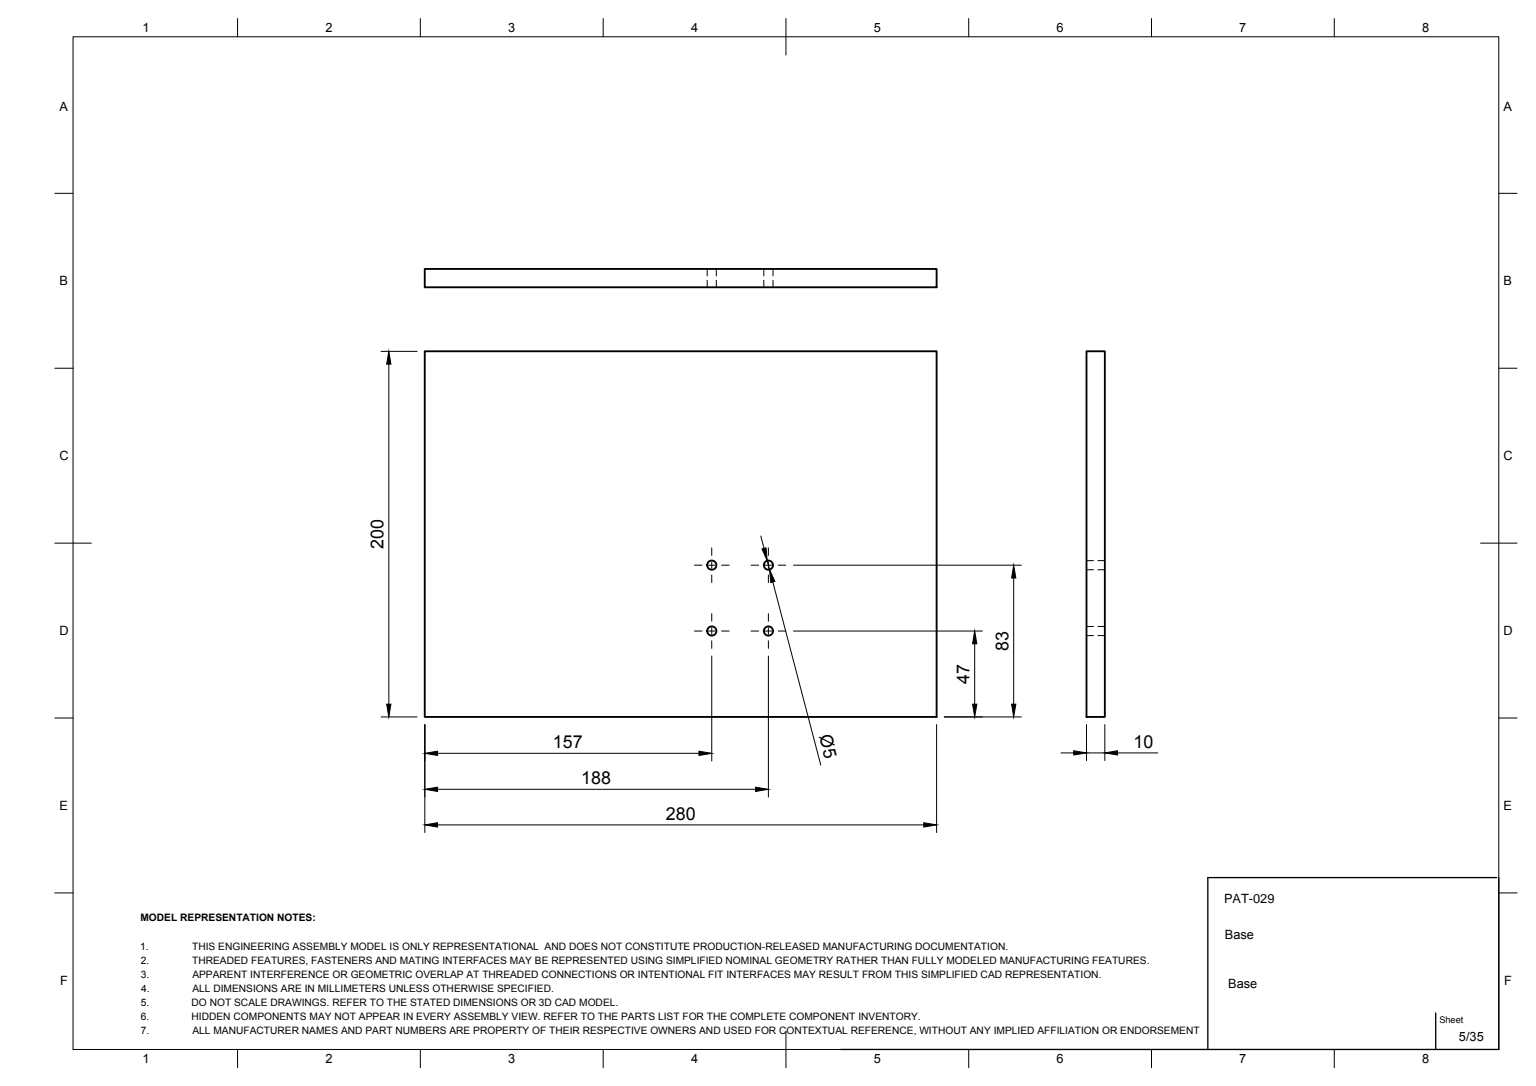
ISO-10303-21;
HEADER;
/* Generated by software containing ST-Developer
 * from STEP Tools, Inc. (www.steptools.com) 
 */

FILE_DESCRIPTION(
/* description */ ('Door-style hinge test fixture with detent'),
/* implementation_level */ '2;1');

FILE_NAME(
/* name */ 'Base.step',
/* time_stamp */ '2026-10-28T03:24:57-07:00',
/* author */ (''),
/* organization */ (''),
/* preprocessor_version */ 'ST-DEVELOPER v20.2',
/* originating_system */ 'Autodesk Translation Framework v15.17.0.0',
/* authorisation */ '');

FILE_SCHEMA (('AUTOMOTIVE_DESIGN { 1 0 10303 214 3 1 1 }'));
ENDSEC;

DATA;
#10=MECHANICAL_DESIGN_GEOMETRIC_PRESENTATION_REPRESENTATION('',(#322),#9813);
#260=SHAPE_REPRESENTATION_RELATIONSHIP('SRR','None',#9937,#291);
#291=ADVANCED_BREP_SHAPE_REPRESENTATION('',(#362),#9780);
#322=STYLED_ITEM('',(#10162),#362);
#362=MANIFOLD_SOLID_BREP('Body1',#4753);
#399=FACE_BOUND('',#957,.T.);
#400=FACE_BOUND('',#958,.T.);
#401=FACE_BOUND('',#959,.T.);
#402=FACE_BOUND('',#960,.T.);
#403=FACE_BOUND('',#962,.T.);
#404=FACE_BOUND('',#963,.T.);
#405=FACE_BOUND('',#964,.T.);
#406=FACE_BOUND('',#965,.T.);
#500=PLANE('',#5153);
#501=PLANE('',#5154);
#502=PLANE('',#5155);
#503=PLANE('',#5156);
#504=PLANE('',#5157);
#505=PLANE('',#5158);
#663=FACE_OUTER_BOUND('',#948,.T.);
#664=FACE_OUTER_BOUND('',#949,.T.);
#665=FACE_OUTER_BOUND('',#950,.T.);
#666=FACE_OUTER_BOUND('',#951,.T.);
#667=FACE_OUTER_BOUND('',#952,.T.);
#668=FACE_OUTER_BOUND('',#953,.T.);
#669=FACE_OUTER_BOUND('',#954,.T.);
#670=FACE_OUTER_BOUND('',#955,.T.);
#671=FACE_OUTER_BOUND('',#956,.T.);
#672=FACE_OUTER_BOUND('',#961,.T.);
#948=EDGE_LOOP('',(#3207,#3208,#3209,#3210));
#949=EDGE_LOOP('',(#3211,#3212,#3213,#3214));
#950=EDGE_LOOP('',(#3215,#3216,#3217,#3218));
#951=EDGE_LOOP('',(#3219,#3220,#3221,#3222));
#952=EDGE_LOOP('',(#3223,#3224,#3225,#3226));
#953=EDGE_LOOP('',(#3227,#3228,#3229,#3230));
#954=EDGE_LOOP('',(#3231,#3232,#3233,#3234));
#955=EDGE_LOOP('',(#3235,#3236,#3237,#3238));
#956=EDGE_LOOP('',(#3239,#3240,#3241,#3242));
#957=EDGE_LOOP('',(#3243));
#958=EDGE_LOOP('',(#3244));
#959=EDGE_LOOP('',(#3245));
#960=EDGE_LOOP('',(#3246));
#961=EDGE_LOOP('',(#3247,#3248,#3249,#3250));
#962=EDGE_LOOP('',(#3251));
#963=EDGE_LOOP('',(#3252));
#964=EDGE_LOOP('',(#3253));
#965=EDGE_LOOP('',(#3254));
#1334=LINE('',#7304,#1654);
#1335=LINE('',#7310,#1655);
#1336=LINE('',#7316,#1656);
#1337=LINE('',#7322,#1657);
#1338=LINE('',#7327,#1658);
#1339=LINE('',#7329,#1659);
#1340=LINE('',#7331,#1660);
#1341=LINE('',#7332,#1661);
#1342=LINE('',#7335,#1662);
#1343=LINE('',#7337,#1663);
#1344=LINE('',#7338,#1664);
#1345=LINE('',#7341,#1665);
#1346=LINE('',#7343,#1666);
#1347=LINE('',#7344,#1667);
#1348=LINE('',#7346,#1668);
#1349=LINE('',#7347,#1669);
#1654=VECTOR('',#5761,0.25);
#1655=VECTOR('',#5768,0.25);
#1656=VECTOR('',#5775,0.25);
#1657=VECTOR('',#5782,0.25);
#1658=VECTOR('',#5787,1.);
#1659=VECTOR('',#5788,1.);
#1660=VECTOR('',#5789,1.);
#1661=VECTOR('',#5790,1.);
#1662=VECTOR('',#5793,1.);
#1663=VECTOR('',#5794,1.);
#1664=VECTOR('',#5795,1.);
#1665=VECTOR('',#5798,1.);
#1666=VECTOR('',#5799,1.);
#1667=VECTOR('',#5800,1.);
#1668=VECTOR('',#5803,1.);
#1669=VECTOR('',#5804,1.);
#1974=CIRCLE('',#5142,0.25);
#1975=CIRCLE('',#5143,0.25);
#1976=CIRCLE('',#5145,0.25);
#1977=CIRCLE('',#5146,0.25);
#1978=CIRCLE('',#5148,0.25);
#1979=CIRCLE('',#5149,0.25);
#1980=CIRCLE('',#5151,0.25);
#1981=CIRCLE('',#5152,0.25);
#2221=VERTEX_POINT('',#7301);
#2222=VERTEX_POINT('',#7303);
#2223=VERTEX_POINT('',#7307);
#2224=VERTEX_POINT('',#7309);
#2225=VERTEX_POINT('',#7313);
#2226=VERTEX_POINT('',#7315);
#2227=VERTEX_POINT('',#7319);
#2228=VERTEX_POINT('',#7321);
#2229=VERTEX_POINT('',#7325);
#2230=VERTEX_POINT('',#7326);
#2231=VERTEX_POINT('',#7328);
#2232=VERTEX_POINT('',#7330);
#2233=VERTEX_POINT('',#7334);
#2234=VERTEX_POINT('',#7336);
#2235=VERTEX_POINT('',#7340);
#2236=VERTEX_POINT('',#7342);
#2620=EDGE_CURVE('',#2221,#2221,#1974,.T.);
#2621=EDGE_CURVE('',#2221,#2222,#1334,.T.);
#2622=EDGE_CURVE('',#2222,#2222,#1975,.T.);
#2623=EDGE_CURVE('',#2223,#2223,#1976,.T.);
#2624=EDGE_CURVE('',#2223,#2224,#1335,.T.);
#2625=EDGE_CURVE('',#2224,#2224,#1977,.T.);
#2626=EDGE_CURVE('',#2225,#2225,#1978,.T.);
#2627=EDGE_CURVE('',#2225,#2226,#1336,.T.);
#2628=EDGE_CURVE('',#2226,#2226,#1979,.T.);
#2629=EDGE_CURVE('',#2227,#2227,#1980,.T.);
#2630=EDGE_CURVE('',#2227,#2228,#1337,.T.);
#2631=EDGE_CURVE('',#2228,#2228,#1981,.T.);
#2632=EDGE_CURVE('',#2229,#2230,#1338,.T.);
#2633=EDGE_CURVE('',#2230,#2231,#1339,.T.);
#2634=EDGE_CURVE('',#2232,#2231,#1340,.T.);
#2635=EDGE_CURVE('',#2229,#2232,#1341,.T.);
#2636=EDGE_CURVE('',#2233,#2229,#1342,.T.);
#2637=EDGE_CURVE('',#2234,#2232,#1343,.T.);
#2638=EDGE_CURVE('',#2233,#2234,#1344,.T.);
#2639=EDGE_CURVE('',#2235,#2233,#1345,.T.);
#2640=EDGE_CURVE('',#2236,#2234,#1346,.T.);
#2641=EDGE_CURVE('',#2235,#2236,#1347,.T.);
#2642=EDGE_CURVE('',#2230,#2235,#1348,.T.);
#2643=EDGE_CURVE('',#2231,#2236,#1349,.T.);
#3207=ORIENTED_EDGE('',*,*,#2620,.F.);
#3208=ORIENTED_EDGE('',*,*,#2621,.T.);
#3209=ORIENTED_EDGE('',*,*,#2622,.F.);
#3210=ORIENTED_EDGE('',*,*,#2621,.F.);
#3211=ORIENTED_EDGE('',*,*,#2623,.F.);
#3212=ORIENTED_EDGE('',*,*,#2624,.T.);
#3213=ORIENTED_EDGE('',*,*,#2625,.F.);
#3214=ORIENTED_EDGE('',*,*,#2624,.F.);
#3215=ORIENTED_EDGE('',*,*,#2626,.F.);
#3216=ORIENTED_EDGE('',*,*,#2627,.T.);
#3217=ORIENTED_EDGE('',*,*,#2628,.F.);
#3218=ORIENTED_EDGE('',*,*,#2627,.F.);
#3219=ORIENTED_EDGE('',*,*,#2629,.F.);
#3220=ORIENTED_EDGE('',*,*,#2630,.T.);
#3221=ORIENTED_EDGE('',*,*,#2631,.F.);
#3222=ORIENTED_EDGE('',*,*,#2630,.F.);
#3223=ORIENTED_EDGE('',*,*,#2632,.T.);
#3224=ORIENTED_EDGE('',*,*,#2633,.T.);
#3225=ORIENTED_EDGE('',*,*,#2634,.F.);
#3226=ORIENTED_EDGE('',*,*,#2635,.F.);
#3227=ORIENTED_EDGE('',*,*,#2636,.T.);
#3228=ORIENTED_EDGE('',*,*,#2635,.T.);
#3229=ORIENTED_EDGE('',*,*,#2637,.F.);
#3230=ORIENTED_EDGE('',*,*,#2638,.F.);
#3231=ORIENTED_EDGE('',*,*,#2639,.T.);
#3232=ORIENTED_EDGE('',*,*,#2638,.T.);
#3233=ORIENTED_EDGE('',*,*,#2640,.F.);
#3234=ORIENTED_EDGE('',*,*,#2641,.F.);
#3235=ORIENTED_EDGE('',*,*,#2642,.T.);
#3236=ORIENTED_EDGE('',*,*,#2641,.T.);
#3237=ORIENTED_EDGE('',*,*,#2643,.F.);
#3238=ORIENTED_EDGE('',*,*,#2633,.F.);
#3239=ORIENTED_EDGE('',*,*,#2643,.T.);
#3240=ORIENTED_EDGE('',*,*,#2640,.T.);
#3241=ORIENTED_EDGE('',*,*,#2637,.T.);
#3242=ORIENTED_EDGE('',*,*,#2634,.T.);
#3243=ORIENTED_EDGE('',*,*,#2622,.T.);
#3244=ORIENTED_EDGE('',*,*,#2625,.T.);
#3245=ORIENTED_EDGE('',*,*,#2628,.T.);
#3246=ORIENTED_EDGE('',*,*,#2631,.T.);
#3247=ORIENTED_EDGE('',*,*,#2642,.F.);
#3248=ORIENTED_EDGE('',*,*,#2632,.F.);
#3249=ORIENTED_EDGE('',*,*,#2636,.F.);
#3250=ORIENTED_EDGE('',*,*,#2639,.F.);
#3251=ORIENTED_EDGE('',*,*,#2620,.T.);
#3252=ORIENTED_EDGE('',*,*,#2623,.T.);
#3253=ORIENTED_EDGE('',*,*,#2626,.T.);
#3254=ORIENTED_EDGE('',*,*,#2629,.T.);
#4381=CYLINDRICAL_SURFACE('',#5141,0.25);
#4382=CYLINDRICAL_SURFACE('',#5144,0.25);
#4383=CYLINDRICAL_SURFACE('',#5147,0.25);
#4384=CYLINDRICAL_SURFACE('',#5150,0.25);
#4468=ADVANCED_FACE('',(#663),#4381,.F.);
#4469=ADVANCED_FACE('',(#664),#4382,.F.);
#4470=ADVANCED_FACE('',(#665),#4383,.F.);
#4471=ADVANCED_FACE('',(#666),#4384,.F.);
#4472=ADVANCED_FACE('',(#667),#500,.T.);
#4473=ADVANCED_FACE('',(#668),#501,.T.);
#4474=ADVANCED_FACE('',(#669),#502,.T.);
#4475=ADVANCED_FACE('',(#670),#503,.T.);
#4476=ADVANCED_FACE('',(#671,#399,#400,#401,#402),#504,.T.);
#4477=ADVANCED_FACE('',(#672,#403,#404,#405,#406),#505,.F.);
#4753=CLOSED_SHELL('',(#4468,#4469,#4470,#4471,#4472,#4473,#4474,#4475,
#4476,#4477));
#5140=AXIS2_PLACEMENT_3D('',#7299,#5755,#5756);
#5141=AXIS2_PLACEMENT_3D('',#7300,#5757,#5758);
#5142=AXIS2_PLACEMENT_3D('',#7302,#5759,#5760);
#5143=AXIS2_PLACEMENT_3D('',#7305,#5762,#5763);
#5144=AXIS2_PLACEMENT_3D('',#7306,#5764,#5765);
#5145=AXIS2_PLACEMENT_3D('',#7308,#5766,#5767);
#5146=AXIS2_PLACEMENT_3D('',#7311,#5769,#5770);
#5147=AXIS2_PLACEMENT_3D('',#7312,#5771,#5772);
#5148=AXIS2_PLACEMENT_3D('',#7314,#5773,#5774);
#5149=AXIS2_PLACEMENT_3D('',#7317,#5776,#5777);
#5150=AXIS2_PLACEMENT_3D('',#7318,#5778,#5779);
#5151=AXIS2_PLACEMENT_3D('',#7320,#5780,#5781);
#5152=AXIS2_PLACEMENT_3D('',#7323,#5783,#5784);
#5153=AXIS2_PLACEMENT_3D('',#7324,#5785,#5786);
#5154=AXIS2_PLACEMENT_3D('',#7333,#5791,#5792);
#5155=AXIS2_PLACEMENT_3D('',#7339,#5796,#5797);
#5156=AXIS2_PLACEMENT_3D('',#7345,#5801,#5802);
#5157=AXIS2_PLACEMENT_3D('',#7348,#5805,#5806);
#5158=AXIS2_PLACEMENT_3D('',#7349,#5807,#5808);
#5755=DIRECTION('axis',(0.,0.,1.));
#5756=DIRECTION('refdir',(1.,0.,0.));
#5757=DIRECTION('center_axis',(0.,0.,1.));
#5758=DIRECTION('ref_axis',(1.,0.,0.));
#5759=DIRECTION('center_axis',(0.,0.,1.));
#5760=DIRECTION('ref_axis',(1.,0.,0.));
#5761=DIRECTION('',(0.,0.,1.));
#5762=DIRECTION('center_axis',(0.,0.,-1.));
#5763=DIRECTION('ref_axis',(1.,0.,0.));
#5764=DIRECTION('center_axis',(0.,0.,1.));
#5765=DIRECTION('ref_axis',(1.,0.,0.));
#5766=DIRECTION('center_axis',(0.,0.,1.));
#5767=DIRECTION('ref_axis',(1.,0.,0.));
#5768=DIRECTION('',(0.,0.,1.));
#5769=DIRECTION('center_axis',(0.,0.,-1.));
#5770=DIRECTION('ref_axis',(1.,0.,0.));
#5771=DIRECTION('center_axis',(0.,0.,1.));
#5772=DIRECTION('ref_axis',(1.,0.,0.));
#5773=DIRECTION('center_axis',(0.,0.,1.));
#5774=DIRECTION('ref_axis',(1.,0.,0.));
#5775=DIRECTION('',(0.,0.,1.));
#5776=DIRECTION('center_axis',(0.,0.,-1.));
#5777=DIRECTION('ref_axis',(1.,0.,0.));
#5778=DIRECTION('center_axis',(0.,0.,1.));
#5779=DIRECTION('ref_axis',(1.,0.,0.));
#5780=DIRECTION('center_axis',(0.,0.,1.));
#5781=DIRECTION('ref_axis',(1.,0.,0.));
#5782=DIRECTION('',(0.,0.,1.));
#5783=DIRECTION('center_axis',(0.,0.,-1.));
#5784=DIRECTION('ref_axis',(1.,0.,0.));
#5785=DIRECTION('center_axis',(0.,1.,0.));
#5786=DIRECTION('ref_axis',(-1.,0.,0.));
#5787=DIRECTION('',(-1.,0.,0.));
#5788=DIRECTION('',(0.,0.,1.));
#5789=DIRECTION('',(-1.,0.,0.));
#5790=DIRECTION('',(0.,0.,1.));
#5791=DIRECTION('center_axis',(1.,0.,0.));
#5792=DIRECTION('ref_axis',(0.,1.,0.));
#5793=DIRECTION('',(0.,1.,0.));
#5794=DIRECTION('',(0.,1.,0.));
#5795=DIRECTION('',(0.,0.,1.));
#5796=DIRECTION('center_axis',(0.,-1.,0.));
#5797=DIRECTION('ref_axis',(1.,0.,0.));
#5798=DIRECTION('',(1.,0.,0.));
#5799=DIRECTION('',(1.,0.,0.));
#5800=DIRECTION('',(0.,0.,1.));
#5801=DIRECTION('center_axis',(-1.,0.,0.));
#5802=DIRECTION('ref_axis',(0.,-1.,0.));
#5803=DIRECTION('',(0.,-1.,0.));
#5804=DIRECTION('',(0.,-1.,0.));
#5805=DIRECTION('center_axis',(0.,0.,1.));
#5806=DIRECTION('ref_axis',(1.,0.,0.));
#5807=DIRECTION('center_axis',(0.,0.,1.));
#5808=DIRECTION('ref_axis',(1.,0.,0.));
#7299=CARTESIAN_POINT('',(0.,0.,0.));
#7300=CARTESIAN_POINT('Origin',(-2.2,-1.8,-1.1));
#7301=CARTESIAN_POINT('',(-2.45,-1.8,-1.));
#7302=CARTESIAN_POINT('Origin',(-2.2,-1.8,-1.));
#7303=CARTESIAN_POINT('',(-2.45,-1.8,0.));
#7304=CARTESIAN_POINT('',(-2.45,-1.8,-1.1));
#7305=CARTESIAN_POINT('Origin',(-2.2,-1.8,0.));
#7306=CARTESIAN_POINT('Origin',(-5.3,1.8,-1.1));
#7307=CARTESIAN_POINT('',(-5.55,1.8,-1.));
#7308=CARTESIAN_POINT('Origin',(-5.3,1.8,-1.));
#7309=CARTESIAN_POINT('',(-5.55,1.8,0.));
#7310=CARTESIAN_POINT('',(-5.55,1.8,-1.1));
#7311=CARTESIAN_POINT('Origin',(-5.3,1.8,0.));
#7312=CARTESIAN_POINT('Origin',(-5.3,-1.8,-1.1));
#7313=CARTESIAN_POINT('',(-5.55,-1.8,-1.));
#7314=CARTESIAN_POINT('Origin',(-5.3,-1.8,-1.));
#7315=CARTESIAN_POINT('',(-5.55,-1.8,0.));
#7316=CARTESIAN_POINT('',(-5.55,-1.8,-1.1));
#7317=CARTESIAN_POINT('Origin',(-5.3,-1.8,0.));
#7318=CARTESIAN_POINT('Origin',(-2.2,1.8,-1.1));
#7319=CARTESIAN_POINT('',(-2.45,1.8,-1.));
#7320=CARTESIAN_POINT('Origin',(-2.2,1.8,-1.));
#7321=CARTESIAN_POINT('',(-2.45,1.8,0.));
#7322=CARTESIAN_POINT('',(-2.45,1.8,-1.1));
#7323=CARTESIAN_POINT('Origin',(-2.2,1.8,0.));
#7324=CARTESIAN_POINT('Origin',(13.5,13.5,-1.));
#7325=CARTESIAN_POINT('',(13.5,13.5,-1.));
#7326=CARTESIAN_POINT('',(-14.5,13.5,-1.));
#7327=CARTESIAN_POINT('',(13.5,13.5,-1.));
#7328=CARTESIAN_POINT('',(-14.5,13.5,0.));
#7329=CARTESIAN_POINT('',(-14.5,13.5,-1.));
#7330=CARTESIAN_POINT('',(13.5,13.5,0.));
#7331=CARTESIAN_POINT('',(13.5,13.5,0.));
#7332=CARTESIAN_POINT('',(13.5,13.5,-1.));
#7333=CARTESIAN_POINT('Origin',(13.5,-6.5,-1.));
#7334=CARTESIAN_POINT('',(13.5,-6.5,-1.));
#7335=CARTESIAN_POINT('',(13.5,-6.5,-1.));
#7336=CARTESIAN_POINT('',(13.5,-6.5,0.));
#7337=CARTESIAN_POINT('',(13.5,-6.5,0.));
#7338=CARTESIAN_POINT('',(13.5,-6.5,-1.));
#7339=CARTESIAN_POINT('Origin',(-14.5,-6.5,-1.));
#7340=CARTESIAN_POINT('',(-14.5,-6.5,-1.));
#7341=CARTESIAN_POINT('',(-14.5,-6.5,-1.));
#7342=CARTESIAN_POINT('',(-14.5,-6.5,0.));
#7343=CARTESIAN_POINT('',(-14.5,-6.5,0.));
#7344=CARTESIAN_POINT('',(-14.5,-6.5,-1.));
#7345=CARTESIAN_POINT('Origin',(-14.5,13.5,-1.));
#7346=CARTESIAN_POINT('',(-14.5,13.5,-1.));
#7347=CARTESIAN_POINT('',(-14.5,13.5,0.));
#7348=CARTESIAN_POINT('Origin',(-0.5,3.5,0.));
#7349=CARTESIAN_POINT('Origin',(-0.5,3.5,-1.));
#9744=UNCERTAINTY_MEASURE_WITH_UNIT(LENGTH_MEASURE(0.001),#9814,
'DISTANCE_ACCURACY_VALUE',
'Maximum model space distance between geometric entities at asserted c
onnectivities');
#9777=UNCERTAINTY_MEASURE_WITH_UNIT(LENGTH_MEASURE(0.001),#9814,
'DISTANCE_ACCURACY_VALUE',
'Maximum model space distance between geometric entities at asserted c
onnectivities');
#9780=(
GEOMETRIC_REPRESENTATION_CONTEXT(3)
GLOBAL_UNCERTAINTY_ASSIGNED_CONTEXT((#9744))
GLOBAL_UNIT_ASSIGNED_CONTEXT((#9814,#9816,#9817))
REPRESENTATION_CONTEXT('','3D')
);
#9813=(
GEOMETRIC_REPRESENTATION_CONTEXT(3)
GLOBAL_UNCERTAINTY_ASSIGNED_CONTEXT((#9777))
GLOBAL_UNIT_ASSIGNED_CONTEXT((#9814,#9816,#9817))
REPRESENTATION_CONTEXT('','3D')
);
#9814=(
LENGTH_UNIT()
NAMED_UNIT(*)
SI_UNIT(.CENTI.,.METRE.)
);
#9816=(
NAMED_UNIT(*)
PLANE_ANGLE_UNIT()
SI_UNIT($,.RADIAN.)
);
#9817=(
NAMED_UNIT(*)
SI_UNIT($,.STERADIAN.)
SOLID_ANGLE_UNIT()
);
#9820=SHAPE_DEFINITION_REPRESENTATION(#9855,#9937);
#9855=PRODUCT_DEFINITION_SHAPE('',$,#9973);
#9937=SHAPE_REPRESENTATION('',(#5140),#9780);
#9970=PRODUCT_DEFINITION_CONTEXT('part definition',#10077,'design');
#9973=PRODUCT_DEFINITION('Base','Base',#10008,#9970);
#10008=PRODUCT_DEFINITION_FORMATION('',$,#10081);
#10077=APPLICATION_CONTEXT(
'Core Data for Automotive Mechanical Design Process');
#10078=PRODUCT_CONTEXT('part definition',#10077,'mechanical');
#10081=PRODUCT('Base','Base','Base',(#10078));
#10156=COLOUR_RGB('Dark Blue',0.08,0.2,0.34);
#10157=FILL_AREA_STYLE_COLOUR('',#10156);
#10158=FILL_AREA_STYLE('',(#10157));
#10159=SURFACE_STYLE_FILL_AREA(#10158);
#10160=SURFACE_SIDE_STYLE('',(#10159));
#10161=SURFACE_STYLE_USAGE(.BOTH.,#10160);
#10162=PRESENTATION_STYLE_ASSIGNMENT((#10161));
ENDSEC;
END-ISO-10303-21;
